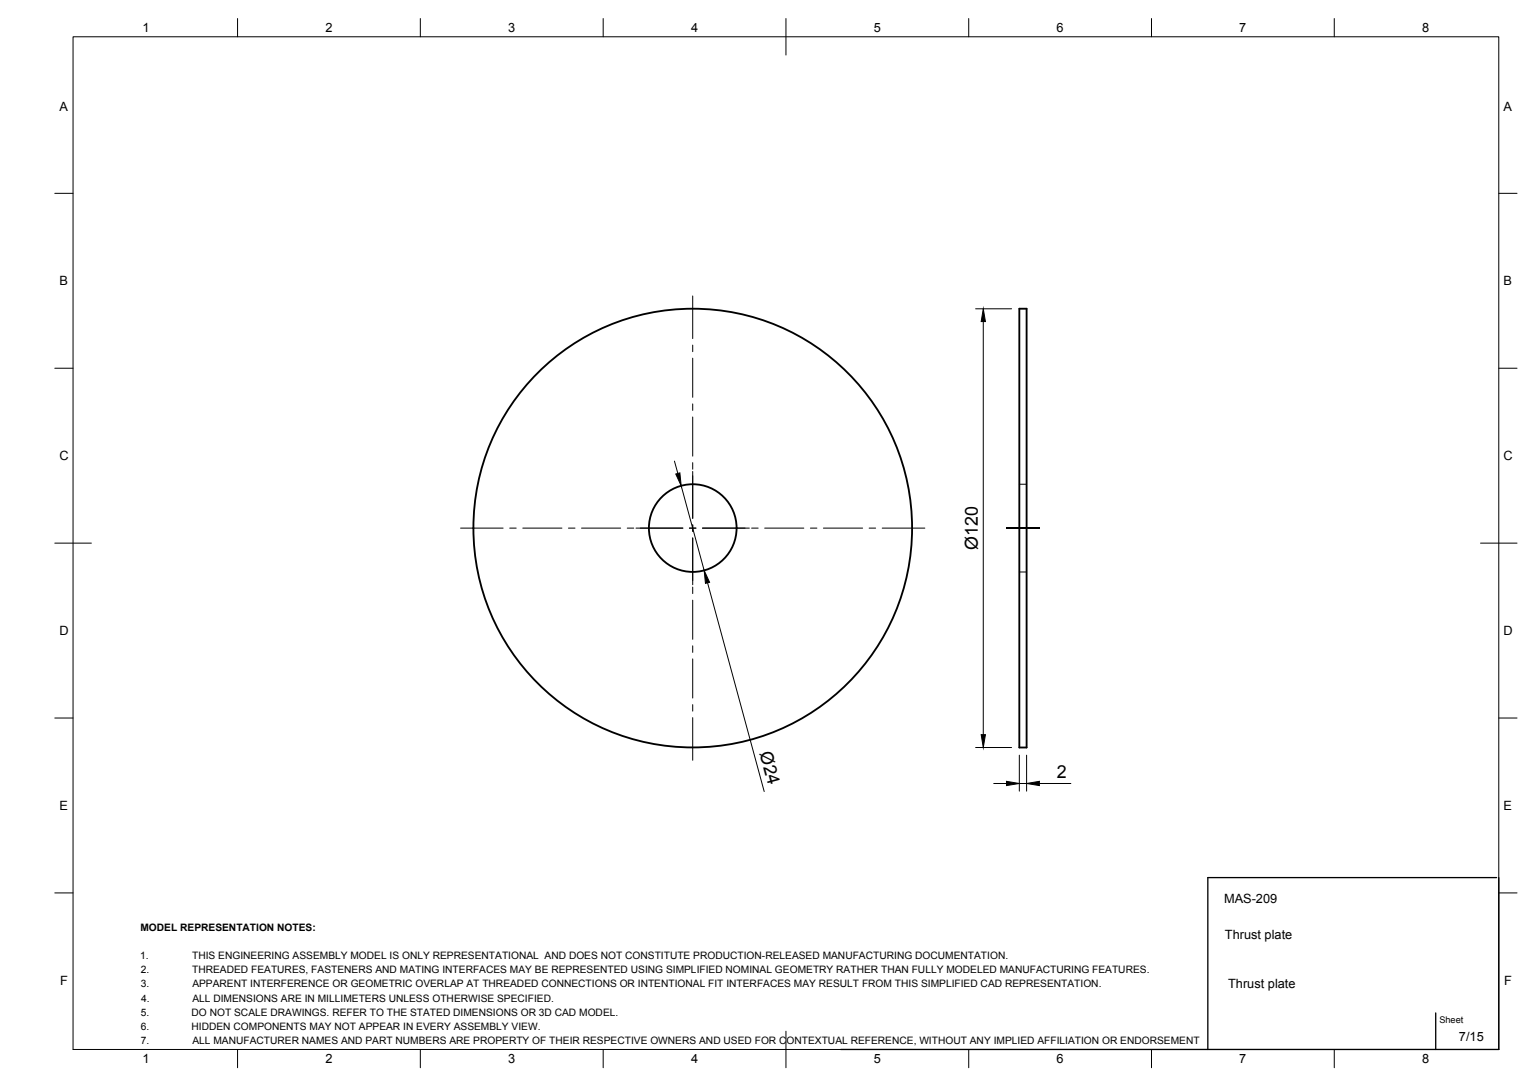
ISO-10303-21;
HEADER;
/* Generated by software containing ST-Developer
 * from STEP Tools, Inc. (www.steptools.com) 
 */

FILE_DESCRIPTION(
/* description */ ('Independent bearing-supported roller-ramp one-way clutch. Six logarit
hmic ramps with plain solid rollers, sprung guided plungers, native Co
il variants, removable shared keepers, rounded parallel key, shaft wit
h complete retaining lips, bronze journal/thrust support and bolted co
vers. Native rotor, roller planar/spin and plunger joints permit manua
l geometric engaged/released inspection. Automatic frictional torque s
witching/contact dynamics are not simulated; no capacity, hardness, fi
t, lubrication, speed, force or life rating. External input driver/cou
pling/anchors outside assembly.'),
/* implementation_level */ '2;1');

FILE_NAME(
/* name */ 'Thrust plate.step',
/* time_stamp */ '2026-11-08T07:04:38-08:00',
/* author */ (''),
/* organization */ (''),
/* preprocessor_version */ 'ST-DEVELOPER v20.2',
/* originating_system */ 'Autodesk Translation Framework v15.17.0.0',
/* authorisation */ '');

FILE_SCHEMA (('AUTOMOTIVE_DESIGN { 1 0 10303 214 3 1 1 }'));
ENDSEC;

DATA;
#10=MECHANICAL_DESIGN_GEOMETRIC_PRESENTATION_REPRESENTATION('',(#306),#99526);
#274=SHAPE_REPRESENTATION_RELATIONSHIP('SRR','None',#99631,#290);
#290=ADVANCED_BREP_SHAPE_REPRESENTATION('',(#322),#99516);
#306=STYLED_ITEM('',(#99717),#322);
#322=MANIFOLD_SOLID_BREP('Body1',#18276);
#414=FACE_BOUND('',#2628,.T.);
#415=FACE_BOUND('',#2630,.T.);
#575=PLANE('',#19553);
#576=PLANE('',#19554);
#1546=FACE_OUTER_BOUND('',#2625,.T.);
#1547=FACE_OUTER_BOUND('',#2626,.T.);
#1548=FACE_OUTER_BOUND('',#2627,.T.);
#1549=FACE_OUTER_BOUND('',#2629,.T.);
#2625=EDGE_LOOP('',(#15936,#15937,#15938,#15939));
#2626=EDGE_LOOP('',(#15940,#15941,#15942,#15943));
#2627=EDGE_LOOP('',(#15944));
#2628=EDGE_LOOP('',(#15945));
#2629=EDGE_LOOP('',(#15946));
#2630=EDGE_LOOP('',(#15947));
#3050=CIRCLE('',#19548,12.);
#3051=CIRCLE('',#19549,12.);
#3052=CIRCLE('',#19551,60.);
#3053=CIRCLE('',#19552,60.);
#5414=LINE('',#94764,#6318);
#5415=LINE('',#94770,#6319);
#6318=VECTOR('',#22755,12.);
#6319=VECTOR('',#22762,60.);
#8065=VERTEX_POINT('',#94761);
#8066=VERTEX_POINT('',#94763);
#8067=VERTEX_POINT('',#94767);
#8068=VERTEX_POINT('',#94769);
#10720=EDGE_CURVE('',#8065,#8065,#3050,.T.);
#10721=EDGE_CURVE('',#8065,#8066,#5414,.T.);
#10722=EDGE_CURVE('',#8066,#8066,#3051,.T.);
#10723=EDGE_CURVE('',#8067,#8067,#3052,.T.);
#10724=EDGE_CURVE('',#8067,#8068,#5415,.T.);
#10725=EDGE_CURVE('',#8068,#8068,#3053,.T.);
#15936=ORIENTED_EDGE('',*,*,#10720,.F.);
#15937=ORIENTED_EDGE('',*,*,#10721,.T.);
#15938=ORIENTED_EDGE('',*,*,#10722,.T.);
#15939=ORIENTED_EDGE('',*,*,#10721,.F.);
#15940=ORIENTED_EDGE('',*,*,#10723,.F.);
#15941=ORIENTED_EDGE('',*,*,#10724,.T.);
#15942=ORIENTED_EDGE('',*,*,#10725,.T.);
#15943=ORIENTED_EDGE('',*,*,#10724,.F.);
#15944=ORIENTED_EDGE('',*,*,#10723,.T.);
#15945=ORIENTED_EDGE('',*,*,#10720,.T.);
#15946=ORIENTED_EDGE('',*,*,#10725,.F.);
#15947=ORIENTED_EDGE('',*,*,#10722,.F.);
#17200=CYLINDRICAL_SURFACE('',#19547,12.);
#17201=CYLINDRICAL_SURFACE('',#19550,60.);
#18144=ADVANCED_FACE('',(#1546),#17200,.F.);
#18145=ADVANCED_FACE('',(#1547),#17201,.T.);
#18146=ADVANCED_FACE('',(#1548,#414),#575,.T.);
#18147=ADVANCED_FACE('',(#1549,#415),#576,.F.);
#18276=CLOSED_SHELL('',(#18144,#18145,#18146,#18147));
#19546=AXIS2_PLACEMENT_3D('',#94759,#22749,#22750);
#19547=AXIS2_PLACEMENT_3D('',#94760,#22751,#22752);
#19548=AXIS2_PLACEMENT_3D('',#94762,#22753,#22754);
#19549=AXIS2_PLACEMENT_3D('',#94765,#22756,#22757);
#19550=AXIS2_PLACEMENT_3D('',#94766,#22758,#22759);
#19551=AXIS2_PLACEMENT_3D('',#94768,#22760,#22761);
#19552=AXIS2_PLACEMENT_3D('',#94771,#22763,#22764);
#19553=AXIS2_PLACEMENT_3D('',#94772,#22765,#22766);
#19554=AXIS2_PLACEMENT_3D('',#94773,#22767,#22768);
#22749=DIRECTION('axis',(0.,0.,1.));
#22750=DIRECTION('refdir',(1.,0.,0.));
#22751=DIRECTION('center_axis',(0.,0.,1.));
#22752=DIRECTION('ref_axis',(1.,0.,0.));
#22753=DIRECTION('center_axis',(0.,0.,-1.));
#22754=DIRECTION('ref_axis',(1.,0.,0.));
#22755=DIRECTION('',(0.,0.,-1.));
#22756=DIRECTION('center_axis',(0.,0.,-1.));
#22757=DIRECTION('ref_axis',(1.,0.,0.));
#22758=DIRECTION('center_axis',(0.,0.,1.));
#22759=DIRECTION('ref_axis',(1.,0.,0.));
#22760=DIRECTION('center_axis',(0.,0.,1.));
#22761=DIRECTION('ref_axis',(1.,0.,0.));
#22762=DIRECTION('',(0.,0.,-1.));
#22763=DIRECTION('center_axis',(0.,0.,1.));
#22764=DIRECTION('ref_axis',(1.,0.,0.));
#22765=DIRECTION('center_axis',(0.,0.,1.));
#22766=DIRECTION('ref_axis',(1.,0.,0.));
#22767=DIRECTION('center_axis',(0.,0.,1.));
#22768=DIRECTION('ref_axis',(1.,0.,0.));
#94759=CARTESIAN_POINT('',(0.,0.,0.));
#94760=CARTESIAN_POINT('Origin',(0.,0.,0.));
#94761=CARTESIAN_POINT('',(-12.,-1.46957615897682E-15,2.));
#94762=CARTESIAN_POINT('Origin',(0.,0.,2.));
#94763=CARTESIAN_POINT('',(-12.,-1.46957615897682E-15,0.));
#94764=CARTESIAN_POINT('',(-12.,-1.46957615897682E-15,0.));
#94765=CARTESIAN_POINT('Origin',(0.,0.,0.));
#94766=CARTESIAN_POINT('Origin',(0.,0.,0.));
#94767=CARTESIAN_POINT('',(-60.,-7.34788079488412E-15,2.));
#94768=CARTESIAN_POINT('Origin',(0.,0.,2.));
#94769=CARTESIAN_POINT('',(-60.,-7.34788079488412E-15,0.));
#94770=CARTESIAN_POINT('',(-60.,-7.34788079488412E-15,0.));
#94771=CARTESIAN_POINT('Origin',(0.,0.,0.));
#94772=CARTESIAN_POINT('Origin',(0.,0.,2.));
#94773=CARTESIAN_POINT('Origin',(0.,0.,0.));
#99498=UNCERTAINTY_MEASURE_WITH_UNIT(LENGTH_MEASURE(0.01),#99527,
'DISTANCE_ACCURACY_VALUE',
'Maximum model space distance between geometric entities at asserted c
onnectivities');
#99508=UNCERTAINTY_MEASURE_WITH_UNIT(LENGTH_MEASURE(0.01),#99527,
'DISTANCE_ACCURACY_VALUE',
'Maximum model space distance between geometric entities at asserted c
onnectivities');
#99516=(
GEOMETRIC_REPRESENTATION_CONTEXT(3)
GLOBAL_UNCERTAINTY_ASSIGNED_CONTEXT((#99498))
GLOBAL_UNIT_ASSIGNED_CONTEXT((#99527,#99529,#99530))
REPRESENTATION_CONTEXT('','3D')
);
#99526=(
GEOMETRIC_REPRESENTATION_CONTEXT(3)
GLOBAL_UNCERTAINTY_ASSIGNED_CONTEXT((#99508))
GLOBAL_UNIT_ASSIGNED_CONTEXT((#99527,#99529,#99530))
REPRESENTATION_CONTEXT('','3D')
);
#99527=(
LENGTH_UNIT()
NAMED_UNIT(*)
SI_UNIT(.MILLI.,.METRE.)
);
#99529=(
NAMED_UNIT(*)
PLANE_ANGLE_UNIT()
SI_UNIT($,.RADIAN.)
);
#99530=(
NAMED_UNIT(*)
SI_UNIT($,.STERADIAN.)
SOLID_ANGLE_UNIT()
);
#99538=SHAPE_DEFINITION_REPRESENTATION(#99555,#99631);
#99555=PRODUCT_DEFINITION_SHAPE('',$,#99649);
#99631=SHAPE_REPRESENTATION('',(#19546),#99516);
#99641=PRODUCT_DEFINITION_CONTEXT('part definition',#99694,'design');
#99649=PRODUCT_DEFINITION('Thrust plate','Thrust plate',#99666,#99641);
#99666=PRODUCT_DEFINITION_FORMATION('',$,#99703);
#99694=APPLICATION_CONTEXT(
'Core Data for Automotive Mechanical Design Process');
#99695=PRODUCT_CONTEXT('part definition',#99694,'mechanical');
#99703=PRODUCT('Thrust plate','Thrust plate',$,(#99695));
#99717=PRESENTATION_STYLE_ASSIGNMENT((#99730));
#99730=SURFACE_STYLE_USAGE(.BOTH.,#99743);
#99743=SURFACE_SIDE_STYLE('',(#99756));
#99756=SURFACE_STYLE_FILL_AREA(#99769);
#99769=FILL_AREA_STYLE('Light gray',(#99782));
#99782=FILL_AREA_STYLE_COLOUR('Light gray',#99795);
#99795=COLOUR_RGB('Light gray',0.725490196078431,0.752941176470588,0.792156862745098);
ENDSEC;
END-ISO-10303-21;
